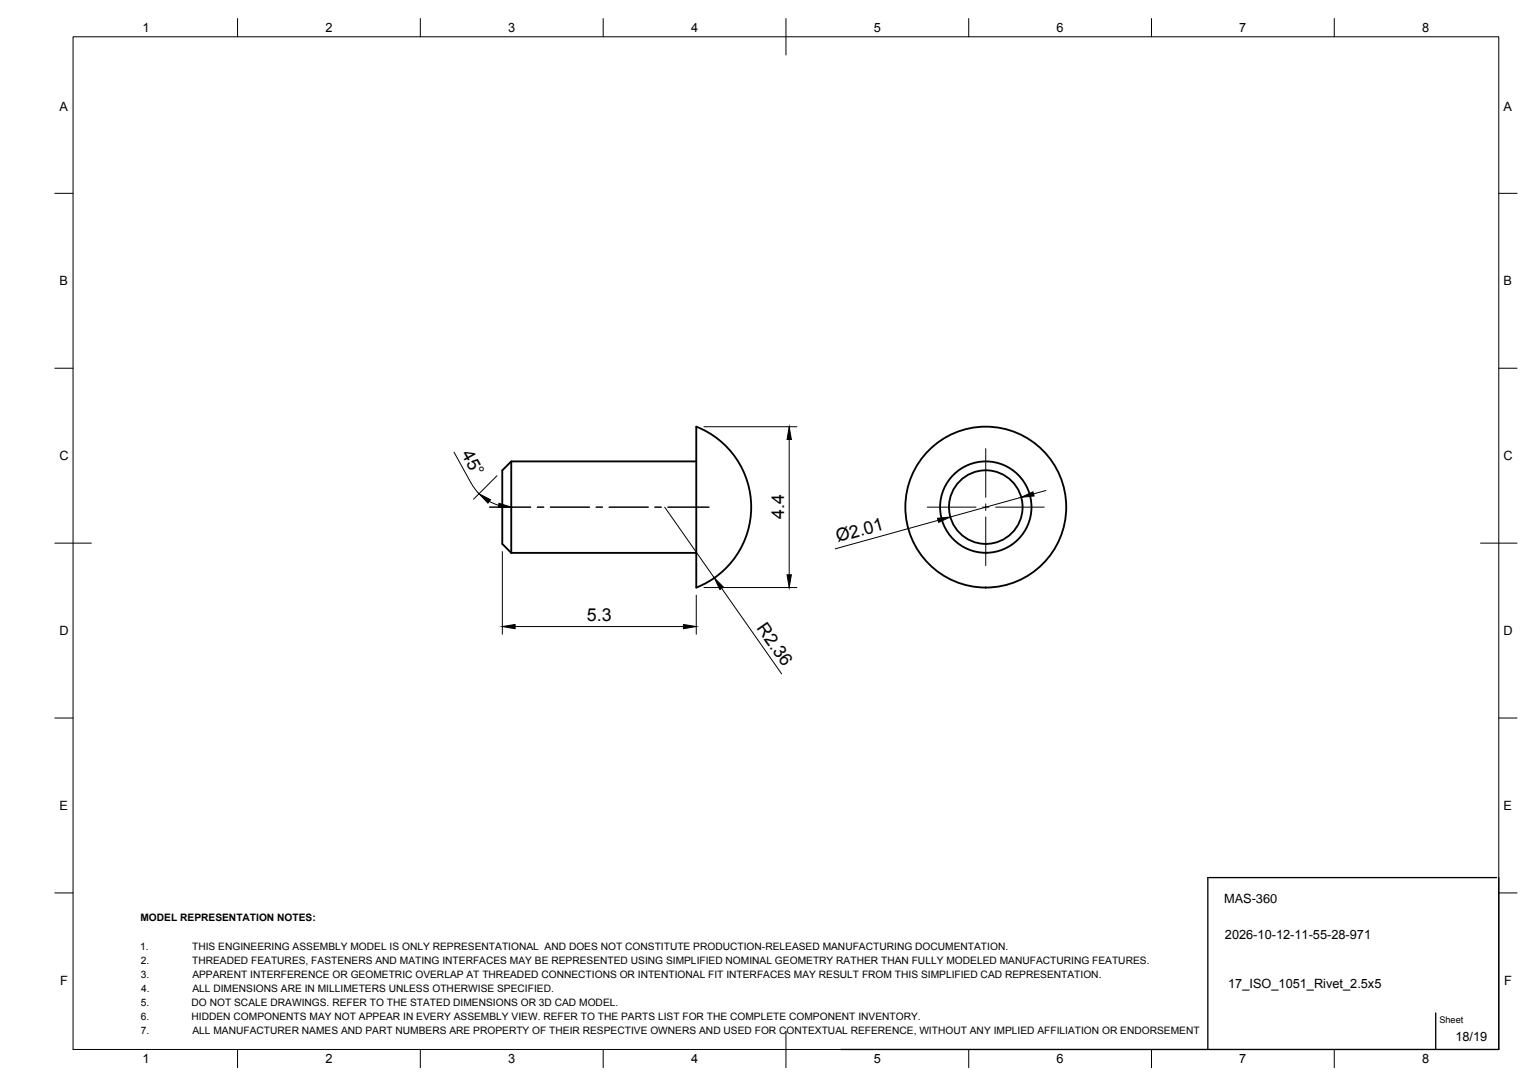
ISO-10303-21;
HEADER;
/* Generated by software containing ST-Developer
 * from STEP Tools, Inc. (www.steptools.com) 
 */

FILE_DESCRIPTION(
/* description */ (''),
/* implementation_level */ '2;1');

FILE_NAME(
/* name */ '17_ISO_1051_Rivet_2.5x5.step',
/* time_stamp */ '2026-11-04T18:53:29-08:00',
/* author */ (''),
/* organization */ (''),
/* preprocessor_version */ 'ST-DEVELOPER v20.2',
/* originating_system */ 'Autodesk Translation Framework v15.17.0.0',
/* authorisation */ '');

FILE_SCHEMA (('AUTOMOTIVE_DESIGN { 1 0 10303 214 3 1 1 }'));
ENDSEC;

DATA;
#10=MECHANICAL_DESIGN_GEOMETRIC_PRESENTATION_REPRESENTATION('',(#1344),#100031);
#226=SPHERICAL_SURFACE('',#22490,2.36333333333333);
#249=CONICAL_SURFACE('',#22496,1.1276,0.785398163397447);
#1179=CIRCLE('',#22491,2.2);
#1180=CIRCLE('',#22493,1.25);
#1181=CIRCLE('',#22495,1.25);
#1182=CIRCLE('',#22497,1.0052);
#1308=SHAPE_REPRESENTATION_RELATIONSHIP('SRR','None',#100118,#1326);
#1326=ADVANCED_BREP_SHAPE_REPRESENTATION('',(#1362),#100030);
#1344=STYLED_ITEM('',(#100204),#1362);
#1362=MANIFOLD_SOLID_BREP('Body1',#20134);
#1692=PLANE('',#22492);
#1693=PLANE('',#22498);
#1810=FACE_BOUND('',#7453,.T.);
#3265=LINE('',#99960,#4552);
#3266=LINE('',#99963,#4553);
#4552=VECTOR('',#28134,1.25);
#4553=VECTOR('',#28137,1.1276);
#5025=CYLINDRICAL_SURFACE('',#22494,1.25);
#6178=FACE_OUTER_BOUND('',#7451,.T.);
#6179=FACE_OUTER_BOUND('',#7452,.T.);
#6180=FACE_OUTER_BOUND('',#7454,.T.);
#6181=FACE_OUTER_BOUND('',#7455,.T.);
#6182=FACE_OUTER_BOUND('',#7456,.T.);
#7451=EDGE_LOOP('',(#18837));
#7452=EDGE_LOOP('',(#18838));
#7453=EDGE_LOOP('',(#18839));
#7454=EDGE_LOOP('',(#18840,#18841,#18842,#18843));
#7455=EDGE_LOOP('',(#18844,#18845,#18846,#18847));
#7456=EDGE_LOOP('',(#18848));
#9920=VERTEX_POINT('',#99952);
#9921=VERTEX_POINT('',#99955);
#9922=VERTEX_POINT('',#99958);
#9923=VERTEX_POINT('',#99962);
#12893=EDGE_CURVE('',#9920,#9920,#1179,.T.);
#12894=EDGE_CURVE('',#9921,#9921,#1180,.T.);
#12895=EDGE_CURVE('',#9922,#9922,#1181,.T.);
#12896=EDGE_CURVE('',#9922,#9921,#3265,.T.);
#12897=EDGE_CURVE('',#9922,#9923,#3266,.T.);
#12898=EDGE_CURVE('',#9923,#9923,#1182,.T.);
#18837=ORIENTED_EDGE('',*,*,#12893,.F.);
#18838=ORIENTED_EDGE('',*,*,#12893,.T.);
#18839=ORIENTED_EDGE('',*,*,#12894,.F.);
#18840=ORIENTED_EDGE('',*,*,#12895,.F.);
#18841=ORIENTED_EDGE('',*,*,#12896,.T.);
#18842=ORIENTED_EDGE('',*,*,#12894,.T.);
#18843=ORIENTED_EDGE('',*,*,#12896,.F.);
#18844=ORIENTED_EDGE('',*,*,#12895,.T.);
#18845=ORIENTED_EDGE('',*,*,#12897,.T.);
#18846=ORIENTED_EDGE('',*,*,#12898,.F.);
#18847=ORIENTED_EDGE('',*,*,#12897,.F.);
#18848=ORIENTED_EDGE('',*,*,#12898,.T.);
#20112=ADVANCED_FACE('',(#6178),#226,.T.);
#20113=ADVANCED_FACE('',(#6179,#1810),#1692,.T.);
#20114=ADVANCED_FACE('',(#6180),#5025,.T.);
#20115=ADVANCED_FACE('',(#6181),#249,.T.);
#20116=ADVANCED_FACE('',(#6182),#1693,.T.);
#20134=CLOSED_SHELL('',(#20112,#20113,#20114,#20115,#20116));
#22489=AXIS2_PLACEMENT_3D('',#99950,#28120,#28121);
#22490=AXIS2_PLACEMENT_3D('',#99951,#28122,#28123);
#22491=AXIS2_PLACEMENT_3D('',#99953,#28124,#28125);
#22492=AXIS2_PLACEMENT_3D('',#99954,#28126,#28127);
#22493=AXIS2_PLACEMENT_3D('',#99956,#28128,#28129);
#22494=AXIS2_PLACEMENT_3D('',#99957,#28130,#28131);
#22495=AXIS2_PLACEMENT_3D('',#99959,#28132,#28133);
#22496=AXIS2_PLACEMENT_3D('',#99961,#28135,#28136);
#22497=AXIS2_PLACEMENT_3D('',#99964,#28138,#28139);
#22498=AXIS2_PLACEMENT_3D('',#99965,#28140,#28141);
#28120=DIRECTION('axis',(0.,0.,1.));
#28121=DIRECTION('refdir',(1.,0.,0.));
#28122=DIRECTION('center_axis',(-9.3953993621311E-17,-8.45359356200646E-19,
1.));
#28123=DIRECTION('ref_axis',(-0.999976174819374,-0.0069028829927877,-4.69787952835825E-17));
#28124=DIRECTION('center_axis',(1.,0.,0.));
#28125=DIRECTION('ref_axis',(0.,0.,-1.));
#28126=DIRECTION('center_axis',(1.,0.,0.));
#28127=DIRECTION('ref_axis',(0.,0.,-1.));
#28128=DIRECTION('center_axis',(1.,0.,0.));
#28129=DIRECTION('ref_axis',(0.,0.,-1.));
#28130=DIRECTION('center_axis',(1.,0.,0.));
#28131=DIRECTION('ref_axis',(0.,1.,0.));
#28132=DIRECTION('center_axis',(1.,0.,0.));
#28133=DIRECTION('ref_axis',(0.,0.,-1.));
#28134=DIRECTION('',(-1.,0.,0.));
#28135=DIRECTION('center_axis',(-1.,0.,0.));
#28136=DIRECTION('ref_axis',(0.,1.,0.));
#28137=DIRECTION('',(0.707106781186548,0.707106781186547,-8.65956056235492E-17));
#28138=DIRECTION('center_axis',(1.,0.,0.));
#28139=DIRECTION('ref_axis',(0.,0.,-1.));
#28140=DIRECTION('center_axis',(1.,0.,0.));
#28141=DIRECTION('ref_axis',(0.,0.,-1.));
#99950=CARTESIAN_POINT('',(0.,0.,0.));
#99951=CARTESIAN_POINT('Origin',(0.863333333333333,5.55111512312578E-16,
0.));
#99952=CARTESIAN_POINT('',(0.,2.2,0.));
#99953=CARTESIAN_POINT('Origin',(0.,0.,0.));
#99954=CARTESIAN_POINT('Origin',(0.,1.25,0.));
#99955=CARTESIAN_POINT('',(0.,-1.25,-1.53080849893419E-16));
#99956=CARTESIAN_POINT('Origin',(0.,0.,0.));
#99957=CARTESIAN_POINT('Origin',(2.5296,0.,0.));
#99958=CARTESIAN_POINT('',(5.0592,-1.25,-1.53080849893419E-16));
#99959=CARTESIAN_POINT('Origin',(5.0592,0.,0.));
#99960=CARTESIAN_POINT('',(2.5296,-1.25,-1.53080849893419E-16));
#99961=CARTESIAN_POINT('Origin',(5.1816,0.,0.));
#99962=CARTESIAN_POINT('',(5.304,-1.0052,-1.23101496250292E-16));
#99963=CARTESIAN_POINT('',(5.1816,-1.1276,1.38091173071856E-16));
#99964=CARTESIAN_POINT('Origin',(5.304,0.,0.));
#99965=CARTESIAN_POINT('Origin',(5.304,0.,0.));
#100010=UNCERTAINTY_MEASURE_WITH_UNIT(LENGTH_MEASURE(0.01),#100032,
'DISTANCE_ACCURACY_VALUE',
'Maximum model space distance between geometric entities at asserted c
onnectivities');
#100011=UNCERTAINTY_MEASURE_WITH_UNIT(LENGTH_MEASURE(0.01),#100032,
'DISTANCE_ACCURACY_VALUE',
'Maximum model space distance between geometric entities at asserted c
onnectivities');
#100030=(
GEOMETRIC_REPRESENTATION_CONTEXT(3)
GLOBAL_UNCERTAINTY_ASSIGNED_CONTEXT((#100010))
GLOBAL_UNIT_ASSIGNED_CONTEXT((#100032,#100034,#100035))
REPRESENTATION_CONTEXT('','3D')
);
#100031=(
GEOMETRIC_REPRESENTATION_CONTEXT(3)
GLOBAL_UNCERTAINTY_ASSIGNED_CONTEXT((#100011))
GLOBAL_UNIT_ASSIGNED_CONTEXT((#100032,#100034,#100035))
REPRESENTATION_CONTEXT('','3D')
);
#100032=(
LENGTH_UNIT()
NAMED_UNIT(*)
SI_UNIT(.MILLI.,.METRE.)
);
#100034=(
NAMED_UNIT(*)
PLANE_ANGLE_UNIT()
SI_UNIT($,.RADIAN.)
);
#100035=(
NAMED_UNIT(*)
SI_UNIT($,.STERADIAN.)
SOLID_ANGLE_UNIT()
);
#100054=SHAPE_DEFINITION_REPRESENTATION(#100073,#100118);
#100073=PRODUCT_DEFINITION_SHAPE('',$,#100138);
#100118=SHAPE_REPRESENTATION('',(#22489),#100030);
#100119=PRODUCT_DEFINITION_CONTEXT('part definition',#100178,'design');
#100138=PRODUCT_DEFINITION('2026-10-12-11-55-28-971',
'17_ISO_1051_Rivet_2.5x5',#100157,#100119);
#100157=PRODUCT_DEFINITION_FORMATION('',$,#100198);
#100178=APPLICATION_CONTEXT(
'Core Data for Automotive Mechanical Design Process');
#100179=PRODUCT_CONTEXT('part definition',#100178,'mechanical');
#100198=PRODUCT('2026-10-12-11-55-28-971','17_ISO_1051_Rivet_2.5x5',$,(#100179));
#100204=PRESENTATION_STYLE_ASSIGNMENT((#100210));
#100210=SURFACE_STYLE_USAGE(.BOTH.,#100216);
#100216=SURFACE_SIDE_STYLE('',(#100222));
#100222=SURFACE_STYLE_FILL_AREA(#100228);
#100228=FILL_AREA_STYLE('Opaque(97,158,199)',(#100234));
#100234=FILL_AREA_STYLE_COLOUR('Opaque(97,158,199)',#100240);
#100240=COLOUR_RGB('Opaque(97,158,199)',0.380392156862745,0.619607843137255,
0.780392156862745);
ENDSEC;
END-ISO-10303-21;
